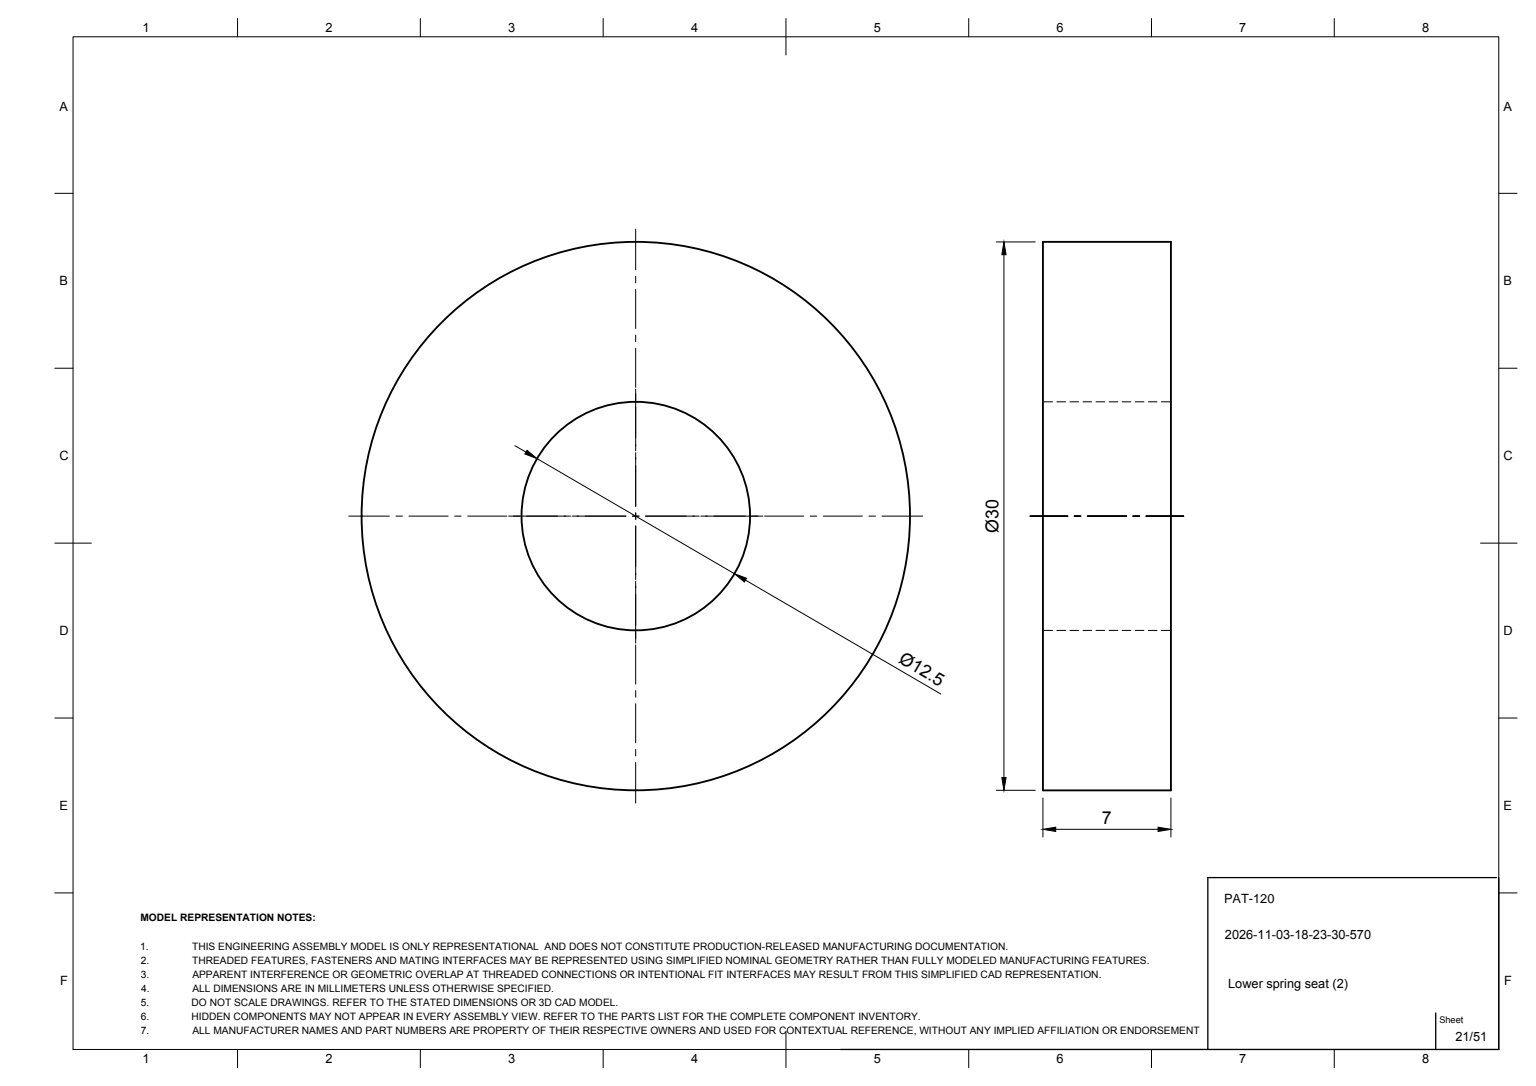
ISO-10303-21;
HEADER;
/* Generated by software containing ST-Developer
 * from STEP Tools, Inc. (www.steptools.com) 
 */

FILE_DESCRIPTION(
/* description */ ('Vibration shaker table dummy'),
/* implementation_level */ '2;1');

FILE_NAME(
/* name */ 'Lower spring seat (2).step',
/* time_stamp */ '2026-10-27T10:55:14-07:00',
/* author */ (''),
/* organization */ (''),
/* preprocessor_version */ 'ST-DEVELOPER v20.2',
/* originating_system */ 'Autodesk Translation Framework v15.17.0.0',
/* authorisation */ '');

FILE_SCHEMA (('AUTOMOTIVE_DESIGN { 1 0 10303 214 3 1 1 }'));
ENDSEC;

DATA;
#10=MECHANICAL_DESIGN_GEOMETRIC_PRESENTATION_REPRESENTATION('',(#702),#22394);
#610=SHAPE_REPRESENTATION_RELATIONSHIP('SRR','None',#22656,#656);
#656=ADVANCED_BREP_SHAPE_REPRESENTATION('',(#748),#22362);
#702=STYLED_ITEM('',(#22961),#748);
#748=MANIFOLD_SOLID_BREP('Body1',#9220);
#903=FACE_BOUND('',#2154,.T.);
#904=FACE_BOUND('',#2156,.T.);
#1166=PLANE('',#10135);
#1167=PLANE('',#10136);
#1525=FACE_OUTER_BOUND('',#2151,.T.);
#1526=FACE_OUTER_BOUND('',#2152,.T.);
#1527=FACE_OUTER_BOUND('',#2153,.T.);
#1528=FACE_OUTER_BOUND('',#2155,.T.);
#2151=EDGE_LOOP('',(#7110,#7111,#7112,#7113));
#2152=EDGE_LOOP('',(#7114,#7115,#7116,#7117));
#2153=EDGE_LOOP('',(#7118));
#2154=EDGE_LOOP('',(#7119));
#2155=EDGE_LOOP('',(#7120));
#2156=EDGE_LOOP('',(#7121));
#2884=LINE('',#17743,#3503);
#2885=LINE('',#17749,#3504);
#3503=VECTOR('',#11954,0.625);
#3504=VECTOR('',#11961,1.5);
#4028=CIRCLE('',#10130,0.625);
#4029=CIRCLE('',#10131,0.625);
#4030=CIRCLE('',#10133,1.5);
#4031=CIRCLE('',#10134,1.5);
#4655=VERTEX_POINT('',#17740);
#4656=VERTEX_POINT('',#17742);
#4657=VERTEX_POINT('',#17746);
#4658=VERTEX_POINT('',#17748);
#5548=EDGE_CURVE('',#4655,#4655,#4028,.T.);
#5549=EDGE_CURVE('',#4655,#4656,#2884,.T.);
#5550=EDGE_CURVE('',#4656,#4656,#4029,.T.);
#5551=EDGE_CURVE('',#4657,#4657,#4030,.T.);
#5552=EDGE_CURVE('',#4657,#4658,#2885,.T.);
#5553=EDGE_CURVE('',#4658,#4658,#4031,.T.);
#7110=ORIENTED_EDGE('',*,*,#5548,.F.);
#7111=ORIENTED_EDGE('',*,*,#5549,.T.);
#7112=ORIENTED_EDGE('',*,*,#5550,.T.);
#7113=ORIENTED_EDGE('',*,*,#5549,.F.);
#7114=ORIENTED_EDGE('',*,*,#5551,.F.);
#7115=ORIENTED_EDGE('',*,*,#5552,.T.);
#7116=ORIENTED_EDGE('',*,*,#5553,.T.);
#7117=ORIENTED_EDGE('',*,*,#5552,.F.);
#7118=ORIENTED_EDGE('',*,*,#5551,.T.);
#7119=ORIENTED_EDGE('',*,*,#5548,.T.);
#7120=ORIENTED_EDGE('',*,*,#5553,.F.);
#7121=ORIENTED_EDGE('',*,*,#5550,.F.);
#8582=CYLINDRICAL_SURFACE('',#10129,0.625);
#8583=CYLINDRICAL_SURFACE('',#10132,1.5);
#8890=ADVANCED_FACE('',(#1525),#8582,.F.);
#8891=ADVANCED_FACE('',(#1526),#8583,.T.);
#8892=ADVANCED_FACE('',(#1527,#903),#1166,.T.);
#8893=ADVANCED_FACE('',(#1528,#904),#1167,.F.);
#9220=CLOSED_SHELL('',(#8890,#8891,#8892,#8893));
#10128=AXIS2_PLACEMENT_3D('',#17738,#11948,#11949);
#10129=AXIS2_PLACEMENT_3D('',#17739,#11950,#11951);
#10130=AXIS2_PLACEMENT_3D('',#17741,#11952,#11953);
#10131=AXIS2_PLACEMENT_3D('',#17744,#11955,#11956);
#10132=AXIS2_PLACEMENT_3D('',#17745,#11957,#11958);
#10133=AXIS2_PLACEMENT_3D('',#17747,#11959,#11960);
#10134=AXIS2_PLACEMENT_3D('',#17750,#11962,#11963);
#10135=AXIS2_PLACEMENT_3D('',#17751,#11964,#11965);
#10136=AXIS2_PLACEMENT_3D('',#17752,#11966,#11967);
#11948=DIRECTION('axis',(0.,0.,1.));
#11949=DIRECTION('refdir',(1.,0.,0.));
#11950=DIRECTION('center_axis',(0.,0.,1.));
#11951=DIRECTION('ref_axis',(1.,0.,0.));
#11952=DIRECTION('center_axis',(0.,0.,-1.));
#11953=DIRECTION('ref_axis',(1.,0.,0.));
#11954=DIRECTION('',(0.,0.,-1.));
#11955=DIRECTION('center_axis',(0.,0.,-1.));
#11956=DIRECTION('ref_axis',(1.,0.,0.));
#11957=DIRECTION('center_axis',(0.,0.,1.));
#11958=DIRECTION('ref_axis',(1.,0.,0.));
#11959=DIRECTION('center_axis',(0.,0.,1.));
#11960=DIRECTION('ref_axis',(1.,0.,0.));
#11961=DIRECTION('',(0.,0.,-1.));
#11962=DIRECTION('center_axis',(0.,0.,1.));
#11963=DIRECTION('ref_axis',(1.,0.,0.));
#11964=DIRECTION('center_axis',(0.,0.,1.));
#11965=DIRECTION('ref_axis',(1.,0.,0.));
#11966=DIRECTION('center_axis',(0.,0.,1.));
#11967=DIRECTION('ref_axis',(1.,0.,0.));
#17738=CARTESIAN_POINT('',(0.,0.,0.));
#17739=CARTESIAN_POINT('Origin',(6.,-4.,1.9));
#17740=CARTESIAN_POINT('',(5.375,-4.,2.6));
#17741=CARTESIAN_POINT('Origin',(6.,-4.,2.6));
#17742=CARTESIAN_POINT('',(5.375,-4.,1.9));
#17743=CARTESIAN_POINT('',(5.375,-4.,1.9));
#17744=CARTESIAN_POINT('Origin',(6.,-4.,1.9));
#17745=CARTESIAN_POINT('Origin',(6.,-4.,1.9));
#17746=CARTESIAN_POINT('',(4.5,-4.,2.6));
#17747=CARTESIAN_POINT('Origin',(6.,-4.,2.6));
#17748=CARTESIAN_POINT('',(4.5,-4.,1.9));
#17749=CARTESIAN_POINT('',(4.5,-4.,1.9));
#17750=CARTESIAN_POINT('Origin',(6.,-4.,1.9));
#17751=CARTESIAN_POINT('Origin',(6.,-4.,2.6));
#17752=CARTESIAN_POINT('Origin',(6.,-4.,1.9));
#22311=UNCERTAINTY_MEASURE_WITH_UNIT(LENGTH_MEASURE(0.001),#22395,
'DISTANCE_ACCURACY_VALUE',
'Maximum model space distance between geometric entities at asserted c
onnectivities');
#22343=UNCERTAINTY_MEASURE_WITH_UNIT(LENGTH_MEASURE(0.001),#22395,
'DISTANCE_ACCURACY_VALUE',
'Maximum model space distance between geometric entities at asserted c
onnectivities');
#22362=(
GEOMETRIC_REPRESENTATION_CONTEXT(3)
GLOBAL_UNCERTAINTY_ASSIGNED_CONTEXT((#22311))
GLOBAL_UNIT_ASSIGNED_CONTEXT((#22395,#22397,#22398))
REPRESENTATION_CONTEXT('','3D')
);
#22394=(
GEOMETRIC_REPRESENTATION_CONTEXT(3)
GLOBAL_UNCERTAINTY_ASSIGNED_CONTEXT((#22343))
GLOBAL_UNIT_ASSIGNED_CONTEXT((#22395,#22397,#22398))
REPRESENTATION_CONTEXT('','3D')
);
#22395=(
LENGTH_UNIT()
NAMED_UNIT(*)
SI_UNIT(.CENTI.,.METRE.)
);
#22397=(
NAMED_UNIT(*)
PLANE_ANGLE_UNIT()
SI_UNIT($,.RADIAN.)
);
#22398=(
NAMED_UNIT(*)
SI_UNIT($,.STERADIAN.)
SOLID_ANGLE_UNIT()
);
#22417=SHAPE_DEFINITION_REPRESENTATION(#22467,#22656);
#22467=PRODUCT_DEFINITION_SHAPE('',$,#22707);
#22656=SHAPE_REPRESENTATION('',(#10128),#22362);
#22688=PRODUCT_DEFINITION_CONTEXT('part definition',#22840,'design');
#22707=PRODUCT_DEFINITION('Lower spring seat (2)','Lower spring seat (2)',
#22757,#22688);
#22757=PRODUCT_DEFINITION_FORMATION('',$,#22860);
#22840=APPLICATION_CONTEXT(
'Core Data for Automotive Mechanical Design Process');
#22841=PRODUCT_CONTEXT('part definition',#22840,'mechanical');
#22860=PRODUCT('Lower spring seat (2)','Lower spring seat (2)',
'Lower spring seat (2)',(#22841));
#22955=COLOUR_RGB('Grey',0.48,0.52,0.57);
#22956=FILL_AREA_STYLE_COLOUR('',#22955);
#22957=FILL_AREA_STYLE('',(#22956));
#22958=SURFACE_STYLE_FILL_AREA(#22957);
#22959=SURFACE_SIDE_STYLE('',(#22958));
#22960=SURFACE_STYLE_USAGE(.BOTH.,#22959);
#22961=PRESENTATION_STYLE_ASSIGNMENT((#22960));
ENDSEC;
END-ISO-10303-21;
